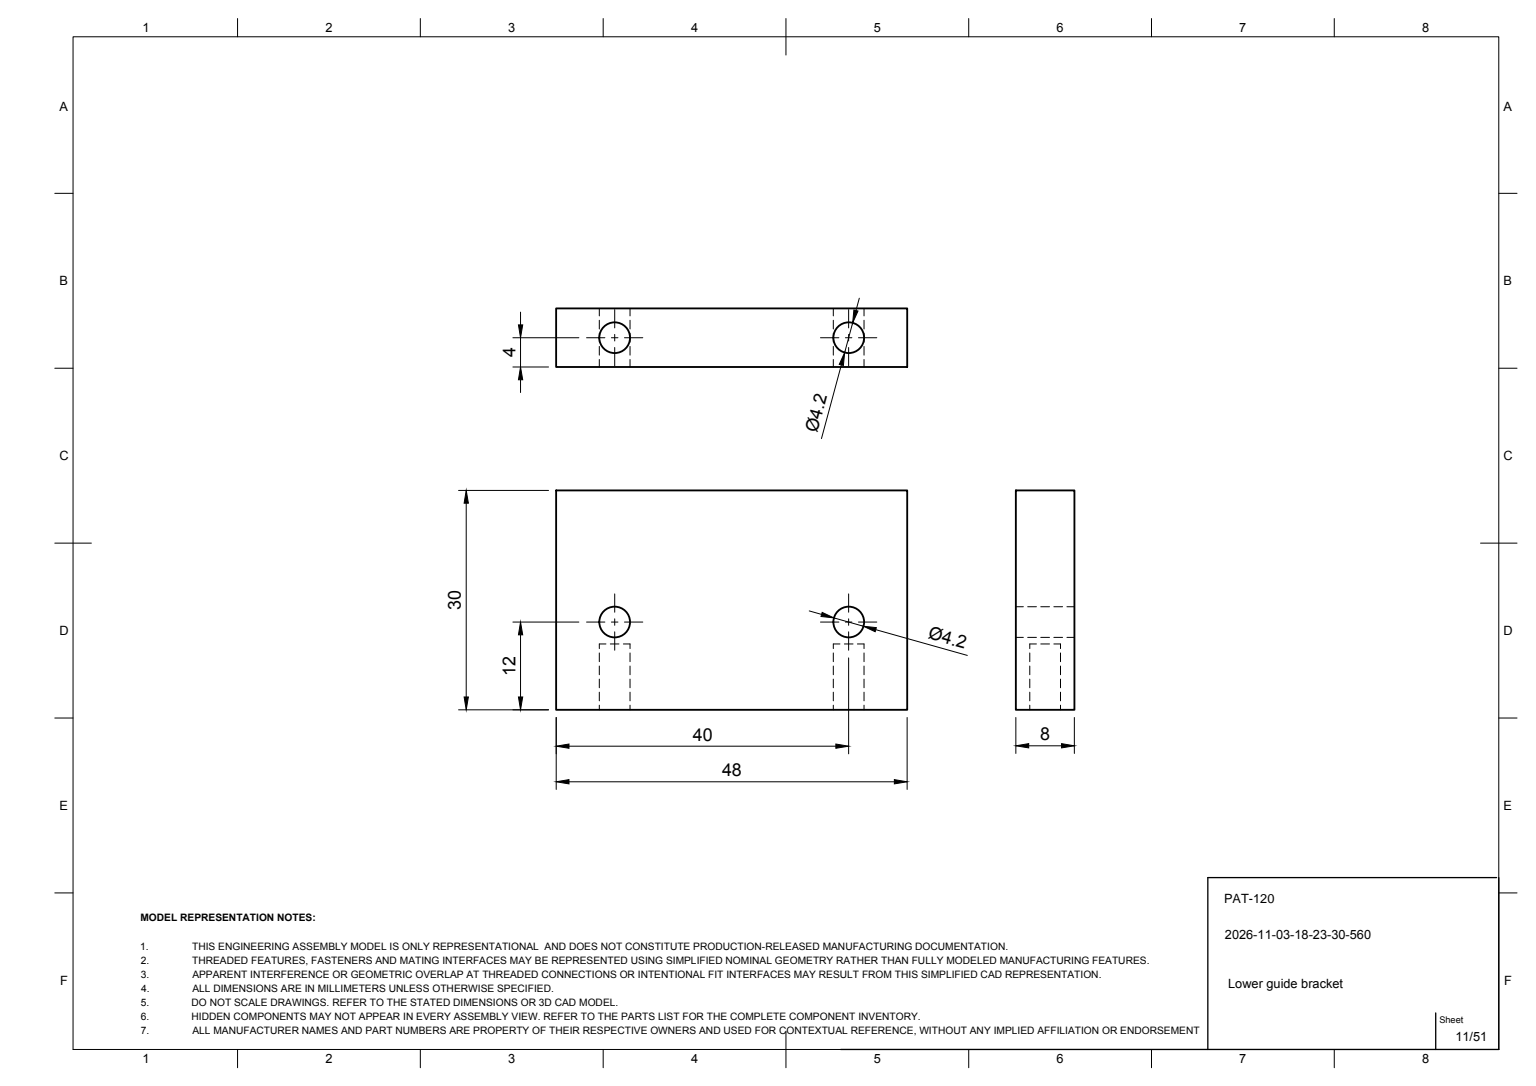
ISO-10303-21;
HEADER;
/* Generated by software containing ST-Developer
 * from STEP Tools, Inc. (www.steptools.com) 
 */

FILE_DESCRIPTION(
/* description */ ('Vibration shaker table dummy'),
/* implementation_level */ '2;1');

FILE_NAME(
/* name */ 'Lower guide bracket.step',
/* time_stamp */ '2026-10-27T10:55:14-07:00',
/* author */ (''),
/* organization */ (''),
/* preprocessor_version */ 'ST-DEVELOPER v20.2',
/* originating_system */ 'Autodesk Translation Framework v15.17.0.0',
/* authorisation */ '');

FILE_SCHEMA (('AUTOMOTIVE_DESIGN { 1 0 10303 214 3 1 1 }'));
ENDSEC;

DATA;
#10=MECHANICAL_DESIGN_GEOMETRIC_PRESENTATION_REPRESENTATION('',(#692),#22394);
#600=SHAPE_REPRESENTATION_RELATIONSHIP('SRR','None',#22646,#646);
#646=ADVANCED_BREP_SHAPE_REPRESENTATION('',(#738),#22352);
#692=STYLED_ITEM('',(#22940),#738);
#738=MANIFOLD_SOLID_BREP('Body1',#9210);
#863=FACE_BOUND('',#2026,.T.);
#864=FACE_BOUND('',#2027,.T.);
#865=FACE_BOUND('',#2030,.T.);
#866=FACE_BOUND('',#2031,.T.);
#867=FACE_BOUND('',#2035,.T.);
#868=FACE_BOUND('',#2036,.T.);
#1104=PLANE('',#9960);
#1105=PLANE('',#9964);
#1106=PLANE('',#9971);
#1107=PLANE('',#9972);
#1108=PLANE('',#9973);
#1109=PLANE('',#9974);
#1110=PLANE('',#9975);
#1111=PLANE('',#9976);
#1433=FACE_OUTER_BOUND('',#2019,.T.);
#1434=FACE_OUTER_BOUND('',#2020,.T.);
#1435=FACE_OUTER_BOUND('',#2021,.T.);
#1436=FACE_OUTER_BOUND('',#2022,.T.);
#1437=FACE_OUTER_BOUND('',#2023,.T.);
#1438=FACE_OUTER_BOUND('',#2024,.T.);
#1439=FACE_OUTER_BOUND('',#2025,.T.);
#1440=FACE_OUTER_BOUND('',#2028,.T.);
#1441=FACE_OUTER_BOUND('',#2029,.T.);
#1442=FACE_OUTER_BOUND('',#2032,.T.);
#1443=FACE_OUTER_BOUND('',#2033,.T.);
#1444=FACE_OUTER_BOUND('',#2034,.T.);
#2019=EDGE_LOOP('',(#6678,#6679,#6680,#6681));
#2020=EDGE_LOOP('',(#6682));
#2021=EDGE_LOOP('',(#6683,#6684,#6685,#6686));
#2022=EDGE_LOOP('',(#6687));
#2023=EDGE_LOOP('',(#6688,#6689,#6690,#6691));
#2024=EDGE_LOOP('',(#6692,#6693,#6694,#6695));
#2025=EDGE_LOOP('',(#6696,#6697,#6698,#6699));
#2026=EDGE_LOOP('',(#6700));
#2027=EDGE_LOOP('',(#6701));
#2028=EDGE_LOOP('',(#6702,#6703,#6704,#6705));
#2029=EDGE_LOOP('',(#6706,#6707,#6708,#6709));
#2030=EDGE_LOOP('',(#6710));
#2031=EDGE_LOOP('',(#6711));
#2032=EDGE_LOOP('',(#6712,#6713,#6714,#6715));
#2033=EDGE_LOOP('',(#6716,#6717,#6718,#6719));
#2034=EDGE_LOOP('',(#6720,#6721,#6722,#6723));
#2035=EDGE_LOOP('',(#6724));
#2036=EDGE_LOOP('',(#6725));
#2742=LINE('',#14414,#3361);
#2743=LINE('',#14421,#3362);
#2744=LINE('',#14428,#3363);
#2745=LINE('',#14434,#3364);
#2746=LINE('',#14439,#3365);
#2747=LINE('',#14441,#3366);
#2748=LINE('',#14443,#3367);
#2749=LINE('',#14444,#3368);
#2750=LINE('',#14447,#3369);
#2751=LINE('',#14449,#3370);
#2752=LINE('',#14450,#3371);
#2753=LINE('',#14453,#3372);
#2754=LINE('',#14455,#3373);
#2755=LINE('',#14456,#3374);
#2756=LINE('',#14458,#3375);
#2757=LINE('',#14459,#3376);
#3361=VECTOR('',#11468,0.21);
#3362=VECTOR('',#11477,0.21);
#3363=VECTOR('',#11486,0.21);
#3364=VECTOR('',#11493,0.21);
#3365=VECTOR('',#11498,1.);
#3366=VECTOR('',#11499,1.);
#3367=VECTOR('',#11500,1.);
#3368=VECTOR('',#11501,1.);
#3369=VECTOR('',#11504,1.);
#3370=VECTOR('',#11505,1.);
#3371=VECTOR('',#11506,1.);
#3372=VECTOR('',#11509,1.);
#3373=VECTOR('',#11510,1.);
#3374=VECTOR('',#11511,1.);
#3375=VECTOR('',#11514,1.);
#3376=VECTOR('',#11515,1.);
#3956=CIRCLE('',#9958,0.21);
#3957=CIRCLE('',#9959,0.21);
#3958=CIRCLE('',#9962,0.21);
#3959=CIRCLE('',#9963,0.21);
#3960=CIRCLE('',#9966,0.21);
#3961=CIRCLE('',#9967,0.21);
#3962=CIRCLE('',#9969,0.21);
#3963=CIRCLE('',#9970,0.21);
#4511=VERTEX_POINT('',#14411);
#4512=VERTEX_POINT('',#14413);
#4513=VERTEX_POINT('',#14418);
#4514=VERTEX_POINT('',#14420);
#4515=VERTEX_POINT('',#14425);
#4516=VERTEX_POINT('',#14427);
#4517=VERTEX_POINT('',#14431);
#4518=VERTEX_POINT('',#14433);
#4519=VERTEX_POINT('',#14437);
#4520=VERTEX_POINT('',#14438);
#4521=VERTEX_POINT('',#14440);
#4522=VERTEX_POINT('',#14442);
#4523=VERTEX_POINT('',#14446);
#4524=VERTEX_POINT('',#14448);
#4525=VERTEX_POINT('',#14452);
#4526=VERTEX_POINT('',#14454);
#5332=EDGE_CURVE('',#4511,#4511,#3956,.T.);
#5333=EDGE_CURVE('',#4511,#4512,#2742,.T.);
#5334=EDGE_CURVE('',#4512,#4512,#3957,.T.);
#5335=EDGE_CURVE('',#4513,#4513,#3958,.T.);
#5336=EDGE_CURVE('',#4513,#4514,#2743,.T.);
#5337=EDGE_CURVE('',#4514,#4514,#3959,.T.);
#5338=EDGE_CURVE('',#4515,#4515,#3960,.T.);
#5339=EDGE_CURVE('',#4515,#4516,#2744,.T.);
#5340=EDGE_CURVE('',#4516,#4516,#3961,.T.);
#5341=EDGE_CURVE('',#4517,#4517,#3962,.T.);
#5342=EDGE_CURVE('',#4517,#4518,#2745,.T.);
#5343=EDGE_CURVE('',#4518,#4518,#3963,.T.);
#5344=EDGE_CURVE('',#4519,#4520,#2746,.T.);
#5345=EDGE_CURVE('',#4520,#4521,#2747,.T.);
#5346=EDGE_CURVE('',#4522,#4521,#2748,.T.);
#5347=EDGE_CURVE('',#4519,#4522,#2749,.T.);
#5348=EDGE_CURVE('',#4523,#4519,#2750,.T.);
#5349=EDGE_CURVE('',#4524,#4522,#2751,.T.);
#5350=EDGE_CURVE('',#4523,#4524,#2752,.T.);
#5351=EDGE_CURVE('',#4525,#4523,#2753,.T.);
#5352=EDGE_CURVE('',#4526,#4524,#2754,.T.);
#5353=EDGE_CURVE('',#4525,#4526,#2755,.T.);
#5354=EDGE_CURVE('',#4520,#4525,#2756,.T.);
#5355=EDGE_CURVE('',#4521,#4526,#2757,.T.);
#6678=ORIENTED_EDGE('',*,*,#5332,.F.);
#6679=ORIENTED_EDGE('',*,*,#5333,.T.);
#6680=ORIENTED_EDGE('',*,*,#5334,.T.);
#6681=ORIENTED_EDGE('',*,*,#5333,.F.);
#6682=ORIENTED_EDGE('',*,*,#5334,.F.);
#6683=ORIENTED_EDGE('',*,*,#5335,.F.);
#6684=ORIENTED_EDGE('',*,*,#5336,.T.);
#6685=ORIENTED_EDGE('',*,*,#5337,.T.);
#6686=ORIENTED_EDGE('',*,*,#5336,.F.);
#6687=ORIENTED_EDGE('',*,*,#5337,.F.);
#6688=ORIENTED_EDGE('',*,*,#5338,.F.);
#6689=ORIENTED_EDGE('',*,*,#5339,.T.);
#6690=ORIENTED_EDGE('',*,*,#5340,.F.);
#6691=ORIENTED_EDGE('',*,*,#5339,.F.);
#6692=ORIENTED_EDGE('',*,*,#5341,.F.);
#6693=ORIENTED_EDGE('',*,*,#5342,.T.);
#6694=ORIENTED_EDGE('',*,*,#5343,.F.);
#6695=ORIENTED_EDGE('',*,*,#5342,.F.);
#6696=ORIENTED_EDGE('',*,*,#5344,.T.);
#6697=ORIENTED_EDGE('',*,*,#5345,.T.);
#6698=ORIENTED_EDGE('',*,*,#5346,.F.);
#6699=ORIENTED_EDGE('',*,*,#5347,.F.);
#6700=ORIENTED_EDGE('',*,*,#5340,.T.);
#6701=ORIENTED_EDGE('',*,*,#5343,.T.);
#6702=ORIENTED_EDGE('',*,*,#5348,.T.);
#6703=ORIENTED_EDGE('',*,*,#5347,.T.);
#6704=ORIENTED_EDGE('',*,*,#5349,.F.);
#6705=ORIENTED_EDGE('',*,*,#5350,.F.);
#6706=ORIENTED_EDGE('',*,*,#5351,.T.);
#6707=ORIENTED_EDGE('',*,*,#5350,.T.);
#6708=ORIENTED_EDGE('',*,*,#5352,.F.);
#6709=ORIENTED_EDGE('',*,*,#5353,.F.);
#6710=ORIENTED_EDGE('',*,*,#5338,.T.);
#6711=ORIENTED_EDGE('',*,*,#5341,.T.);
#6712=ORIENTED_EDGE('',*,*,#5354,.T.);
#6713=ORIENTED_EDGE('',*,*,#5353,.T.);
#6714=ORIENTED_EDGE('',*,*,#5355,.F.);
#6715=ORIENTED_EDGE('',*,*,#5345,.F.);
#6716=ORIENTED_EDGE('',*,*,#5355,.T.);
#6717=ORIENTED_EDGE('',*,*,#5352,.T.);
#6718=ORIENTED_EDGE('',*,*,#5349,.T.);
#6719=ORIENTED_EDGE('',*,*,#5346,.T.);
#6720=ORIENTED_EDGE('',*,*,#5354,.F.);
#6721=ORIENTED_EDGE('',*,*,#5344,.F.);
#6722=ORIENTED_EDGE('',*,*,#5348,.F.);
#6723=ORIENTED_EDGE('',*,*,#5351,.F.);
#6724=ORIENTED_EDGE('',*,*,#5332,.T.);
#6725=ORIENTED_EDGE('',*,*,#5335,.T.);
#8554=CYLINDRICAL_SURFACE('',#9957,0.21);
#8555=CYLINDRICAL_SURFACE('',#9961,0.21);
#8556=CYLINDRICAL_SURFACE('',#9965,0.21);
#8557=CYLINDRICAL_SURFACE('',#9968,0.21);
#8798=ADVANCED_FACE('',(#1433),#8554,.F.);
#8799=ADVANCED_FACE('',(#1434),#1104,.F.);
#8800=ADVANCED_FACE('',(#1435),#8555,.F.);
#8801=ADVANCED_FACE('',(#1436),#1105,.F.);
#8802=ADVANCED_FACE('',(#1437),#8556,.F.);
#8803=ADVANCED_FACE('',(#1438),#8557,.F.);
#8804=ADVANCED_FACE('',(#1439,#863,#864),#1106,.T.);
#8805=ADVANCED_FACE('',(#1440),#1107,.T.);
#8806=ADVANCED_FACE('',(#1441,#865,#866),#1108,.T.);
#8807=ADVANCED_FACE('',(#1442),#1109,.T.);
#8808=ADVANCED_FACE('',(#1443),#1110,.T.);
#8809=ADVANCED_FACE('',(#1444,#867,#868),#1111,.F.);
#9210=CLOSED_SHELL('',(#8798,#8799,#8800,#8801,#8802,#8803,#8804,#8805,
#8806,#8807,#8808,#8809));
#9956=AXIS2_PLACEMENT_3D('',#14409,#11462,#11463);
#9957=AXIS2_PLACEMENT_3D('',#14410,#11464,#11465);
#9958=AXIS2_PLACEMENT_3D('',#14412,#11466,#11467);
#9959=AXIS2_PLACEMENT_3D('',#14415,#11469,#11470);
#9960=AXIS2_PLACEMENT_3D('',#14416,#11471,#11472);
#9961=AXIS2_PLACEMENT_3D('',#14417,#11473,#11474);
#9962=AXIS2_PLACEMENT_3D('',#14419,#11475,#11476);
#9963=AXIS2_PLACEMENT_3D('',#14422,#11478,#11479);
#9964=AXIS2_PLACEMENT_3D('',#14423,#11480,#11481);
#9965=AXIS2_PLACEMENT_3D('',#14424,#11482,#11483);
#9966=AXIS2_PLACEMENT_3D('',#14426,#11484,#11485);
#9967=AXIS2_PLACEMENT_3D('',#14429,#11487,#11488);
#9968=AXIS2_PLACEMENT_3D('',#14430,#11489,#11490);
#9969=AXIS2_PLACEMENT_3D('',#14432,#11491,#11492);
#9970=AXIS2_PLACEMENT_3D('',#14435,#11494,#11495);
#9971=AXIS2_PLACEMENT_3D('',#14436,#11496,#11497);
#9972=AXIS2_PLACEMENT_3D('',#14445,#11502,#11503);
#9973=AXIS2_PLACEMENT_3D('',#14451,#11507,#11508);
#9974=AXIS2_PLACEMENT_3D('',#14457,#11512,#11513);
#9975=AXIS2_PLACEMENT_3D('',#14460,#11516,#11517);
#9976=AXIS2_PLACEMENT_3D('',#14461,#11518,#11519);
#11462=DIRECTION('axis',(0.,0.,1.));
#11463=DIRECTION('refdir',(1.,0.,0.));
#11464=DIRECTION('center_axis',(0.,0.,1.));
#11465=DIRECTION('ref_axis',(1.,0.,0.));
#11466=DIRECTION('center_axis',(0.,0.,1.));
#11467=DIRECTION('ref_axis',(1.,0.,0.));
#11468=DIRECTION('',(0.,0.,1.));
#11469=DIRECTION('center_axis',(0.,0.,1.));
#11470=DIRECTION('ref_axis',(1.,0.,0.));
#11471=DIRECTION('center_axis',(0.,0.,1.));
#11472=DIRECTION('ref_axis',(1.,0.,0.));
#11473=DIRECTION('center_axis',(0.,0.,1.));
#11474=DIRECTION('ref_axis',(1.,0.,0.));
#11475=DIRECTION('center_axis',(0.,0.,1.));
#11476=DIRECTION('ref_axis',(1.,0.,0.));
#11477=DIRECTION('',(0.,0.,1.));
#11478=DIRECTION('center_axis',(0.,0.,1.));
#11479=DIRECTION('ref_axis',(1.,0.,0.));
#11480=DIRECTION('center_axis',(0.,0.,1.));
#11481=DIRECTION('ref_axis',(1.,0.,0.));
#11482=DIRECTION('center_axis',(0.,1.,0.));
#11483=DIRECTION('ref_axis',(1.,0.,0.));
#11484=DIRECTION('center_axis',(0.,1.,0.));
#11485=DIRECTION('ref_axis',(1.,0.,0.));
#11486=DIRECTION('',(0.,1.,0.));
#11487=DIRECTION('center_axis',(0.,-1.,0.));
#11488=DIRECTION('ref_axis',(1.,0.,0.));
#11489=DIRECTION('center_axis',(0.,1.,0.));
#11490=DIRECTION('ref_axis',(1.,0.,0.));
#11491=DIRECTION('center_axis',(0.,1.,0.));
#11492=DIRECTION('ref_axis',(1.,0.,0.));
#11493=DIRECTION('',(0.,1.,0.));
#11494=DIRECTION('center_axis',(0.,-1.,0.));
#11495=DIRECTION('ref_axis',(1.,0.,0.));
#11496=DIRECTION('center_axis',(0.,1.,0.));
#11497=DIRECTION('ref_axis',(-1.,0.,0.));
#11498=DIRECTION('',(-1.,0.,0.));
#11499=DIRECTION('',(0.,0.,1.));
#11500=DIRECTION('',(-1.,0.,0.));
#11501=DIRECTION('',(0.,0.,1.));
#11502=DIRECTION('center_axis',(1.,0.,0.));
#11503=DIRECTION('ref_axis',(0.,1.,0.));
#11504=DIRECTION('',(0.,1.,0.));
#11505=DIRECTION('',(0.,1.,0.));
#11506=DIRECTION('',(0.,0.,1.));
#11507=DIRECTION('center_axis',(0.,-1.,0.));
#11508=DIRECTION('ref_axis',(1.,0.,0.));
#11509=DIRECTION('',(1.,0.,0.));
#11510=DIRECTION('',(1.,0.,0.));
#11511=DIRECTION('',(0.,0.,1.));
#11512=DIRECTION('center_axis',(-1.,0.,0.));
#11513=DIRECTION('ref_axis',(0.,-1.,0.));
#11514=DIRECTION('',(0.,-1.,0.));
#11515=DIRECTION('',(0.,-1.,0.));
#11516=DIRECTION('center_axis',(0.,0.,1.));
#11517=DIRECTION('ref_axis',(1.,0.,0.));
#11518=DIRECTION('center_axis',(0.,0.,1.));
#11519=DIRECTION('ref_axis',(1.,0.,0.));
#14409=CARTESIAN_POINT('',(0.,0.,0.));
#14410=CARTESIAN_POINT('Origin',(-7.6,-1.3,-0.1));
#14411=CARTESIAN_POINT('',(-7.81,-1.3,0.));
#14412=CARTESIAN_POINT('Origin',(-7.6,-1.3,0.));
#14413=CARTESIAN_POINT('',(-7.81,-1.3,0.9));
#14414=CARTESIAN_POINT('',(-7.81,-1.3,-0.1));
#14415=CARTESIAN_POINT('Origin',(-7.6,-1.3,0.9));
#14416=CARTESIAN_POINT('Origin',(-7.6,-1.3,0.9));
#14417=CARTESIAN_POINT('Origin',(-4.4,-1.3,-0.1));
#14418=CARTESIAN_POINT('',(-4.61,-1.3,0.));
#14419=CARTESIAN_POINT('Origin',(-4.4,-1.3,0.));
#14420=CARTESIAN_POINT('',(-4.61,-1.3,0.9));
#14421=CARTESIAN_POINT('',(-4.61,-1.3,-0.1));
#14422=CARTESIAN_POINT('Origin',(-4.4,-1.3,0.9));
#14423=CARTESIAN_POINT('Origin',(-4.4,-1.3,0.9));
#14424=CARTESIAN_POINT('Origin',(-7.6,-1.8,1.2));
#14425=CARTESIAN_POINT('',(-7.81,-1.7,1.2));
#14426=CARTESIAN_POINT('Origin',(-7.6,-1.7,1.2));
#14427=CARTESIAN_POINT('',(-7.81,-0.9,1.2));
#14428=CARTESIAN_POINT('',(-7.81,-1.8,1.2));
#14429=CARTESIAN_POINT('Origin',(-7.6,-0.9,1.2));
#14430=CARTESIAN_POINT('Origin',(-4.4,-1.8,1.2));
#14431=CARTESIAN_POINT('',(-4.61,-1.7,1.2));
#14432=CARTESIAN_POINT('Origin',(-4.4,-1.7,1.2));
#14433=CARTESIAN_POINT('',(-4.61,-0.9,1.2));
#14434=CARTESIAN_POINT('',(-4.61,-1.8,1.2));
#14435=CARTESIAN_POINT('Origin',(-4.4,-0.9,1.2));
#14436=CARTESIAN_POINT('Origin',(-3.6,-0.9,0.));
#14437=CARTESIAN_POINT('',(-3.6,-0.9,0.));
#14438=CARTESIAN_POINT('',(-8.4,-0.9,0.));
#14439=CARTESIAN_POINT('',(-3.6,-0.9,0.));
#14440=CARTESIAN_POINT('',(-8.4,-0.9,3.));
#14441=CARTESIAN_POINT('',(-8.4,-0.9,0.));
#14442=CARTESIAN_POINT('',(-3.6,-0.9,3.));
#14443=CARTESIAN_POINT('',(-3.6,-0.9,3.));
#14444=CARTESIAN_POINT('',(-3.6,-0.9,0.));
#14445=CARTESIAN_POINT('Origin',(-3.6,-1.7,0.));
#14446=CARTESIAN_POINT('',(-3.6,-1.7,0.));
#14447=CARTESIAN_POINT('',(-3.6,-1.7,0.));
#14448=CARTESIAN_POINT('',(-3.6,-1.7,3.));
#14449=CARTESIAN_POINT('',(-3.6,-1.7,3.));
#14450=CARTESIAN_POINT('',(-3.6,-1.7,0.));
#14451=CARTESIAN_POINT('Origin',(-8.4,-1.7,0.));
#14452=CARTESIAN_POINT('',(-8.4,-1.7,0.));
#14453=CARTESIAN_POINT('',(-8.4,-1.7,0.));
#14454=CARTESIAN_POINT('',(-8.4,-1.7,3.));
#14455=CARTESIAN_POINT('',(-8.4,-1.7,3.));
#14456=CARTESIAN_POINT('',(-8.4,-1.7,0.));
#14457=CARTESIAN_POINT('Origin',(-8.4,-0.9,0.));
#14458=CARTESIAN_POINT('',(-8.4,-0.9,0.));
#14459=CARTESIAN_POINT('',(-8.4,-0.9,3.));
#14460=CARTESIAN_POINT('Origin',(-6.,-1.3,3.));
#14461=CARTESIAN_POINT('Origin',(-6.,-1.3,0.));
#22301=UNCERTAINTY_MEASURE_WITH_UNIT(LENGTH_MEASURE(0.001),#22395,
'DISTANCE_ACCURACY_VALUE',
'Maximum model space distance between geometric entities at asserted c
onnectivities');
#22343=UNCERTAINTY_MEASURE_WITH_UNIT(LENGTH_MEASURE(0.001),#22395,
'DISTANCE_ACCURACY_VALUE',
'Maximum model space distance between geometric entities at asserted c
onnectivities');
#22352=(
GEOMETRIC_REPRESENTATION_CONTEXT(3)
GLOBAL_UNCERTAINTY_ASSIGNED_CONTEXT((#22301))
GLOBAL_UNIT_ASSIGNED_CONTEXT((#22395,#22397,#22398))
REPRESENTATION_CONTEXT('','3D')
);
#22394=(
GEOMETRIC_REPRESENTATION_CONTEXT(3)
GLOBAL_UNCERTAINTY_ASSIGNED_CONTEXT((#22343))
GLOBAL_UNIT_ASSIGNED_CONTEXT((#22395,#22397,#22398))
REPRESENTATION_CONTEXT('','3D')
);
#22395=(
LENGTH_UNIT()
NAMED_UNIT(*)
SI_UNIT(.CENTI.,.METRE.)
);
#22397=(
NAMED_UNIT(*)
PLANE_ANGLE_UNIT()
SI_UNIT($,.RADIAN.)
);
#22398=(
NAMED_UNIT(*)
SI_UNIT($,.STERADIAN.)
SOLID_ANGLE_UNIT()
);
#22407=SHAPE_DEFINITION_REPRESENTATION(#22457,#22646);
#22457=PRODUCT_DEFINITION_SHAPE('',$,#22697);
#22646=SHAPE_REPRESENTATION('',(#9956),#22352);
#22688=PRODUCT_DEFINITION_CONTEXT('part definition',#22840,'design');
#22697=PRODUCT_DEFINITION('Lower guide bracket','Lower guide bracket',#22747,
#22688);
#22747=PRODUCT_DEFINITION_FORMATION('',$,#22850);
#22840=APPLICATION_CONTEXT(
'Core Data for Automotive Mechanical Design Process');
#22841=PRODUCT_CONTEXT('part definition',#22840,'mechanical');
#22850=PRODUCT('Lower guide bracket','Lower guide bracket',
'Lower guide bracket',(#22841));
#22934=COLOUR_RGB('Dark Blue',0.08,0.2,0.34);
#22935=FILL_AREA_STYLE_COLOUR('',#22934);
#22936=FILL_AREA_STYLE('',(#22935));
#22937=SURFACE_STYLE_FILL_AREA(#22936);
#22938=SURFACE_SIDE_STYLE('',(#22937));
#22939=SURFACE_STYLE_USAGE(.BOTH.,#22938);
#22940=PRESENTATION_STYLE_ASSIGNMENT((#22939));
ENDSEC;
END-ISO-10303-21;
